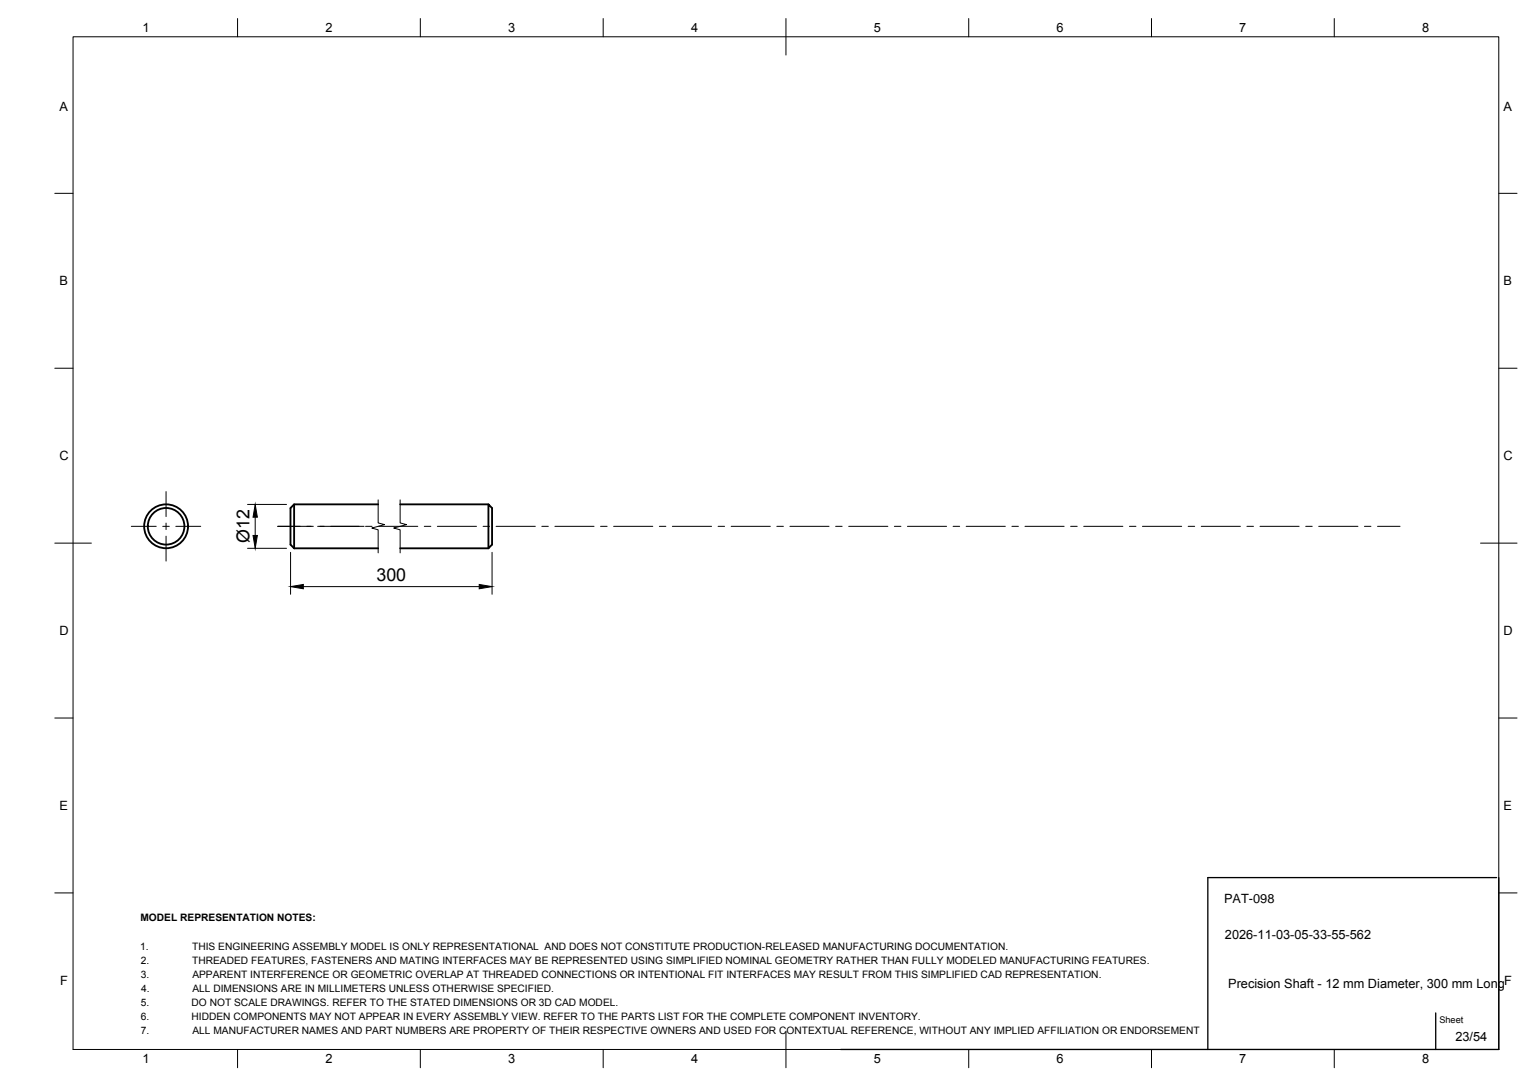
ISO-10303-21;
HEADER;
/* Generated by software containing ST-Developer
 * from STEP Tools, Inc. (www.steptools.com) 
 */

FILE_DESCRIPTION(
/* description */ ('Spring compression tester'),
/* implementation_level */ '2;1');

FILE_NAME(
/* name */ 'Precision Shaft - 12 mm Diameter, 300 mm Long.step',
/* time_stamp */ '2026-10-28T03:24:11-07:00',
/* author */ (''),
/* organization */ (''),
/* preprocessor_version */ 'ST-DEVELOPER v20.2',
/* originating_system */ 'Autodesk Translation Framework v15.17.0.0',
/* authorisation */ '');

FILE_SCHEMA (('AUTOMOTIVE_DESIGN { 1 0 10303 214 3 1 1 }'));
ENDSEC;

DATA;
#10=MECHANICAL_DESIGN_GEOMETRIC_PRESENTATION_REPRESENTATION('',(#1124),#43521);
#945=CONICAL_SURFACE('',#19921,0.55,0.785398163397448);
#946=CONICAL_SURFACE('',#19927,0.55,0.785398163397441);
#1004=SHAPE_REPRESENTATION_RELATIONSHIP('SRR','None',#43816,#1064);
#1064=ADVANCED_BREP_SHAPE_REPRESENTATION('',(#1199),#43476);
#1124=STYLED_ITEM('',(#44202),#1199);
#1199=MANIFOLD_SOLID_BREP('Body1',#18561);
#1859=PLANE('',#19926);
#1860=PLANE('',#19929);
#2552=FACE_OUTER_BOUND('',#3791,.T.);
#2553=FACE_OUTER_BOUND('',#3792,.T.);
#2554=FACE_OUTER_BOUND('',#3793,.T.);
#2555=FACE_OUTER_BOUND('',#3794,.T.);
#2556=FACE_OUTER_BOUND('',#3795,.T.);
#3791=EDGE_LOOP('',(#13921,#13922,#13923,#13924));
#3792=EDGE_LOOP('',(#13925,#13926,#13927,#13928));
#3793=EDGE_LOOP('',(#13929));
#3794=EDGE_LOOP('',(#13930,#13931,#13932,#13933));
#3795=EDGE_LOOP('',(#13934));
#5226=LINE('',#28281,#6658);
#5227=LINE('',#28286,#6659);
#5228=LINE('',#28291,#6660);
#6658=VECTOR('',#23094,0.55);
#6659=VECTOR('',#23101,0.6);
#6660=VECTOR('',#23108,0.55);
#7702=CIRCLE('',#19922,0.6);
#7703=CIRCLE('',#19923,0.5);
#7704=CIRCLE('',#19925,0.6);
#7705=CIRCLE('',#19928,0.5);
#8704=VERTEX_POINT('',#28278);
#8705=VERTEX_POINT('',#28280);
#8706=VERTEX_POINT('',#28284);
#8707=VERTEX_POINT('',#28289);
#10625=EDGE_CURVE('',#8704,#8704,#7702,.T.);
#10626=EDGE_CURVE('',#8704,#8705,#5226,.T.);
#10627=EDGE_CURVE('',#8705,#8705,#7703,.T.);
#10628=EDGE_CURVE('',#8706,#8706,#7704,.T.);
#10629=EDGE_CURVE('',#8706,#8704,#5227,.T.);
#10630=EDGE_CURVE('',#8707,#8707,#7705,.T.);
#10631=EDGE_CURVE('',#8707,#8706,#5228,.T.);
#13921=ORIENTED_EDGE('',*,*,#10625,.T.);
#13922=ORIENTED_EDGE('',*,*,#10626,.T.);
#13923=ORIENTED_EDGE('',*,*,#10627,.T.);
#13924=ORIENTED_EDGE('',*,*,#10626,.F.);
#13925=ORIENTED_EDGE('',*,*,#10628,.F.);
#13926=ORIENTED_EDGE('',*,*,#10629,.T.);
#13927=ORIENTED_EDGE('',*,*,#10625,.F.);
#13928=ORIENTED_EDGE('',*,*,#10629,.F.);
#13929=ORIENTED_EDGE('',*,*,#10627,.F.);
#13930=ORIENTED_EDGE('',*,*,#10630,.T.);
#13931=ORIENTED_EDGE('',*,*,#10631,.T.);
#13932=ORIENTED_EDGE('',*,*,#10628,.T.);
#13933=ORIENTED_EDGE('',*,*,#10631,.F.);
#13934=ORIENTED_EDGE('',*,*,#10630,.F.);
#17217=CYLINDRICAL_SURFACE('',#19924,0.6);
#17876=ADVANCED_FACE('',(#2552),#945,.T.);
#17877=ADVANCED_FACE('',(#2553),#17217,.T.);
#17878=ADVANCED_FACE('',(#2554),#1859,.F.);
#17879=ADVANCED_FACE('',(#2555),#946,.T.);
#17880=ADVANCED_FACE('',(#2556),#1860,.T.);
#18561=CLOSED_SHELL('',(#17876,#17877,#17878,#17879,#17880));
#19920=AXIS2_PLACEMENT_3D('',#28276,#23088,#23089);
#19921=AXIS2_PLACEMENT_3D('',#28277,#23090,#23091);
#19922=AXIS2_PLACEMENT_3D('',#28279,#23092,#23093);
#19923=AXIS2_PLACEMENT_3D('',#28282,#23095,#23096);
#19924=AXIS2_PLACEMENT_3D('',#28283,#23097,#23098);
#19925=AXIS2_PLACEMENT_3D('',#28285,#23099,#23100);
#19926=AXIS2_PLACEMENT_3D('',#28287,#23102,#23103);
#19927=AXIS2_PLACEMENT_3D('',#28288,#23104,#23105);
#19928=AXIS2_PLACEMENT_3D('',#28290,#23106,#23107);
#19929=AXIS2_PLACEMENT_3D('',#28292,#23109,#23110);
#23088=DIRECTION('axis',(0.,0.,1.));
#23089=DIRECTION('refdir',(1.,0.,0.));
#23090=DIRECTION('center_axis',(1.,0.,0.));
#23091=DIRECTION('ref_axis',(0.,0.,-1.));
#23092=DIRECTION('center_axis',(-1.,0.,0.));
#23093=DIRECTION('ref_axis',(0.,0.,-1.));
#23094=DIRECTION('',(-0.707106781186548,8.65956056235493E-17,-0.707106781186547));
#23095=DIRECTION('center_axis',(1.,0.,0.));
#23096=DIRECTION('ref_axis',(0.,0.,-1.));
#23097=DIRECTION('center_axis',(1.,0.,0.));
#23098=DIRECTION('ref_axis',(0.,0.,-1.));
#23099=DIRECTION('center_axis',(1.,0.,0.));
#23100=DIRECTION('ref_axis',(0.,0.,-1.));
#23101=DIRECTION('',(-1.,0.,0.));
#23102=DIRECTION('center_axis',(1.,0.,0.));
#23103=DIRECTION('ref_axis',(0.,0.,-1.));
#23104=DIRECTION('center_axis',(-1.,0.,0.));
#23105=DIRECTION('ref_axis',(0.,0.,-1.));
#23106=DIRECTION('center_axis',(-1.,0.,0.));
#23107=DIRECTION('ref_axis',(0.,0.,-1.));
#23108=DIRECTION('',(-0.707106781186553,-8.65956056235487E-17,0.707106781186542));
#23109=DIRECTION('center_axis',(1.,0.,0.));
#23110=DIRECTION('ref_axis',(0.,0.,-1.));
#28276=CARTESIAN_POINT('',(0.,0.,0.));
#28277=CARTESIAN_POINT('Origin',(0.05,0.,0.));
#28278=CARTESIAN_POINT('',(0.1,7.34788079488412E-17,0.6));
#28279=CARTESIAN_POINT('Origin',(0.1,0.,0.));
#28280=CARTESIAN_POINT('',(0.,-6.12323399573677E-17,0.5));
#28281=CARTESIAN_POINT('',(0.05,-6.73555739531044E-17,0.55));
#28282=CARTESIAN_POINT('Origin',(0.,0.,0.));
#28283=CARTESIAN_POINT('Origin',(0.,0.,0.));
#28284=CARTESIAN_POINT('',(29.9,-7.34788079488412E-17,0.6));
#28285=CARTESIAN_POINT('Origin',(29.9,0.,0.));
#28286=CARTESIAN_POINT('',(0.,-7.34788079488412E-17,0.6));
#28287=CARTESIAN_POINT('Origin',(0.,0.,0.));
#28288=CARTESIAN_POINT('Origin',(29.95,0.,0.));
#28289=CARTESIAN_POINT('',(30.,6.12323399573677E-17,0.5));
#28290=CARTESIAN_POINT('Origin',(30.,0.,0.));
#28291=CARTESIAN_POINT('',(29.95,-6.73555739531044E-17,0.55));
#28292=CARTESIAN_POINT('Origin',(30.,0.,0.));
#43408=UNCERTAINTY_MEASURE_WITH_UNIT(LENGTH_MEASURE(0.001),#43522,
'DISTANCE_ACCURACY_VALUE',
'Maximum model space distance between geometric entities at asserted c
onnectivities');
#43453=UNCERTAINTY_MEASURE_WITH_UNIT(LENGTH_MEASURE(0.001),#43522,
'DISTANCE_ACCURACY_VALUE',
'Maximum model space distance between geometric entities at asserted c
onnectivities');
#43476=(
GEOMETRIC_REPRESENTATION_CONTEXT(3)
GLOBAL_UNCERTAINTY_ASSIGNED_CONTEXT((#43408))
GLOBAL_UNIT_ASSIGNED_CONTEXT((#43522,#43524,#43525))
REPRESENTATION_CONTEXT('','3D')
);
#43521=(
GEOMETRIC_REPRESENTATION_CONTEXT(3)
GLOBAL_UNCERTAINTY_ASSIGNED_CONTEXT((#43453))
GLOBAL_UNIT_ASSIGNED_CONTEXT((#43522,#43524,#43525))
REPRESENTATION_CONTEXT('','3D')
);
#43522=(
LENGTH_UNIT()
NAMED_UNIT(*)
SI_UNIT(.CENTI.,.METRE.)
);
#43524=(
NAMED_UNIT(*)
PLANE_ANGLE_UNIT()
SI_UNIT($,.RADIAN.)
);
#43525=(
NAMED_UNIT(*)
SI_UNIT($,.STERADIAN.)
SOLID_ANGLE_UNIT()
);
#43548=SHAPE_DEFINITION_REPRESENTATION(#43615,#43816);
#43615=PRODUCT_DEFINITION_SHAPE('',$,#43884);
#43816=SHAPE_REPRESENTATION('',(#19920),#43476);
#43861=PRODUCT_DEFINITION_CONTEXT('part definition',#44064,'design');
#43884=PRODUCT_DEFINITION(
'Precision Shaft - 12 mm Diameter, 300 mm Long',
'Precision Shaft - 12 mm Diameter, 300 mm Long',#43951,#43861);
#43951=PRODUCT_DEFINITION_FORMATION('',$,#44088);
#44064=APPLICATION_CONTEXT(
'Core Data for Automotive Mechanical Design Process');
#44065=PRODUCT_CONTEXT('part definition',#44064,'mechanical');
#44088=PRODUCT('Precision Shaft - 12 mm Diameter, 300 mm Long',
'Precision Shaft - 12 mm Diameter, 300 mm Long',
'Precision Shaft - 12 mm Diameter, 300 mm Long',(#44065));
#44196=COLOUR_RGB('Grey',0.48,0.52,0.57);
#44197=FILL_AREA_STYLE_COLOUR('',#44196);
#44198=FILL_AREA_STYLE('',(#44197));
#44199=SURFACE_STYLE_FILL_AREA(#44198);
#44200=SURFACE_SIDE_STYLE('',(#44199));
#44201=SURFACE_STYLE_USAGE(.BOTH.,#44200);
#44202=PRESENTATION_STYLE_ASSIGNMENT((#44201));
ENDSEC;
END-ISO-10303-21;
